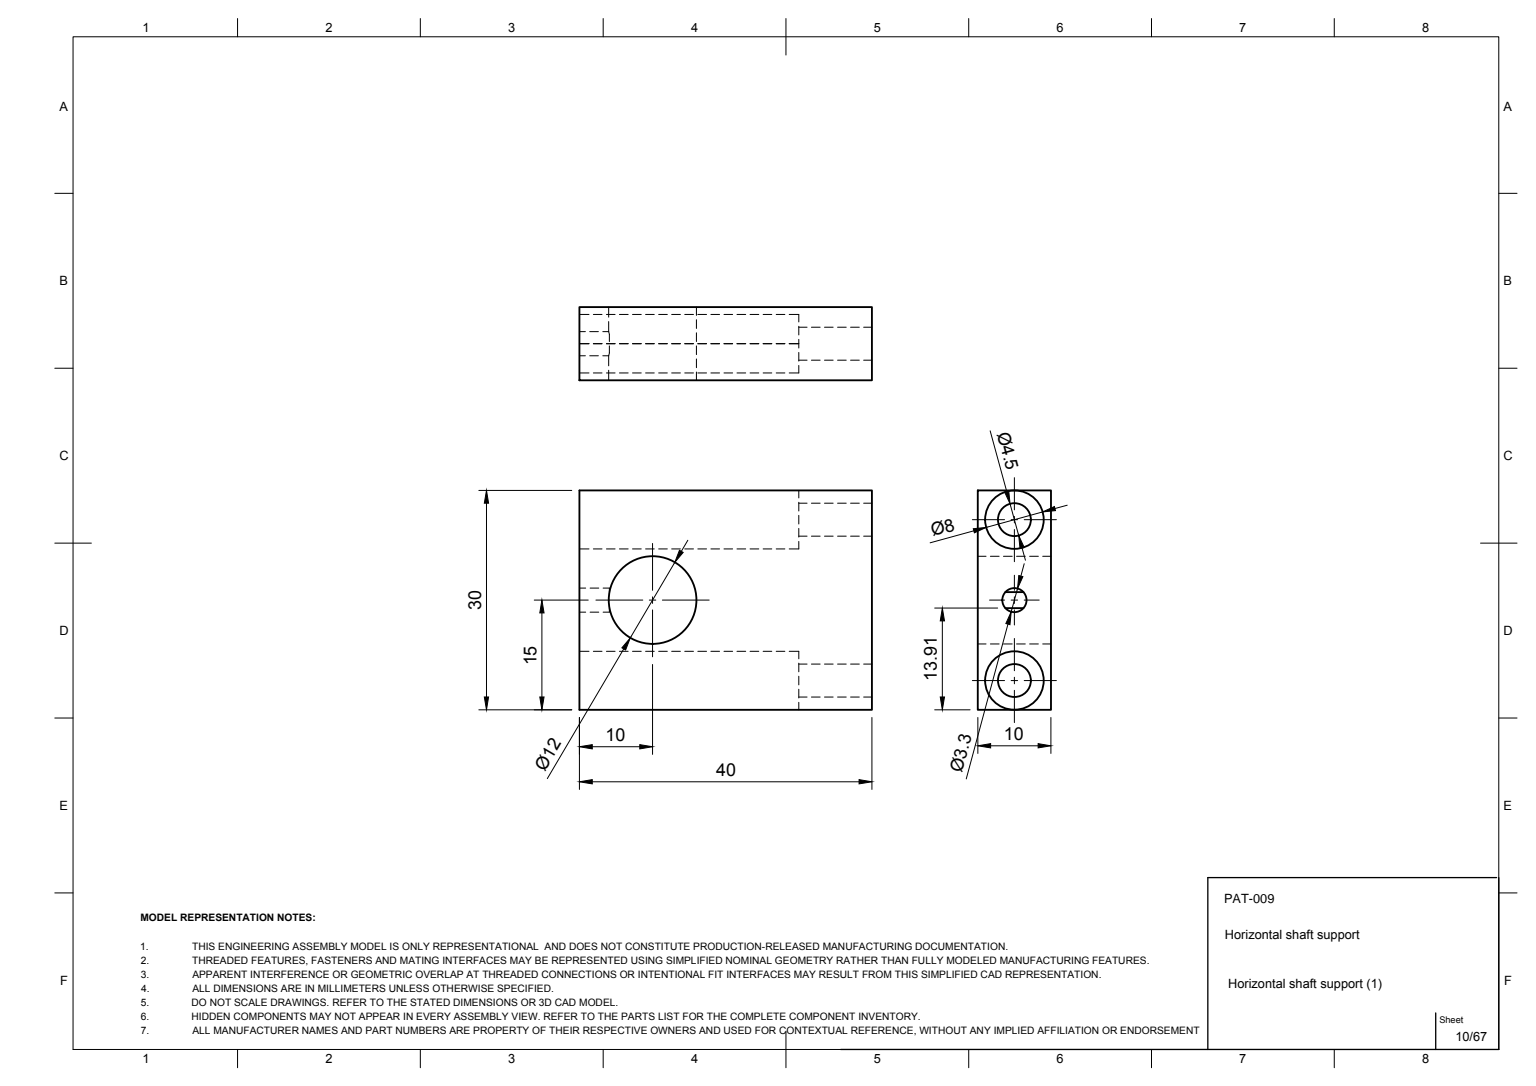
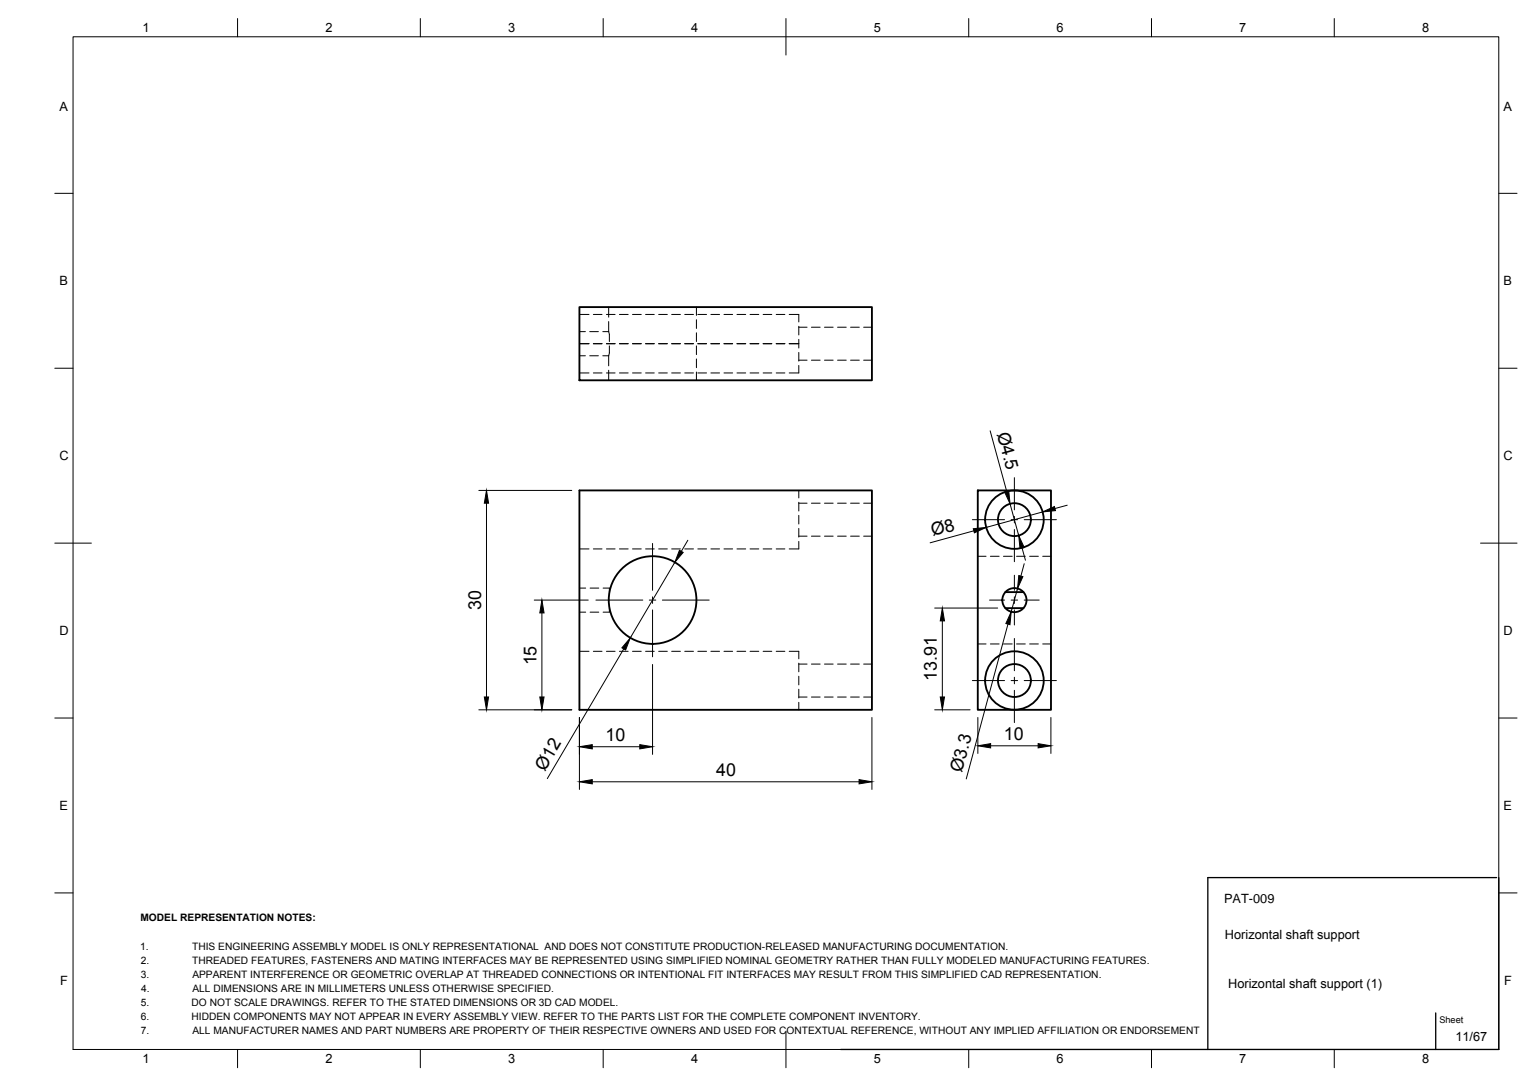
ISO-10303-21;
HEADER;
/* Generated by software containing ST-Developer
 * from STEP Tools, Inc. (www.steptools.com) 
 */

FILE_DESCRIPTION(
/* description */ ('Bell-crank linkage with push rods'),
/* implementation_level */ '2;1');

FILE_NAME(
/* name */ 'Horizontal shaft support.step',
/* time_stamp */ '2026-10-28T03:25:15-07:00',
/* author */ (''),
/* organization */ (''),
/* preprocessor_version */ 'ST-DEVELOPER v20.2',
/* originating_system */ 'Autodesk Translation Framework v15.17.0.0',
/* authorisation */ '');

FILE_SCHEMA (('AUTOMOTIVE_DESIGN { 1 0 10303 214 3 1 1 }'));
ENDSEC;

DATA;
#10=MECHANICAL_DESIGN_GEOMETRIC_PRESENTATION_REPRESENTATION('',(#609),#16678);
#461=B_SPLINE_CURVE_WITH_KNOTS('',3,(#13994,#13995,#13996,#13997,#13998,
#13999),.UNSPECIFIED.,.F.,.F.,(4,2,4),(0.635430324955934,0.687528937234029,
0.750024497760675),.UNSPECIFIED.);
#462=B_SPLINE_CURVE_WITH_KNOTS('',3,(#14003,#14004,#14005,#14006,#14007,
#14008),.UNSPECIFIED.,.F.,.F.,(4,2,4),(0.250008165920225,0.312503726446871,
0.364602338724967),.UNSPECIFIED.);
#463=B_SPLINE_CURVE_WITH_KNOTS('',3,(#14009,#14010,#14011,#14012,#14013,
#14014),.UNSPECIFIED.,.F.,.F.,(4,2,4),(0.135413993115484,0.187512605393579,
0.250008165920225),.UNSPECIFIED.);
#464=B_SPLINE_CURVE_WITH_KNOTS('',3,(#14015,#14016,#14017,#14018,#14019,
#14020),.UNSPECIFIED.,.F.,.F.,(4,2,4),(0.750024497760675,0.81252005828732,
0.864618670565416),.UNSPECIFIED.);
#501=SHAPE_REPRESENTATION_RELATIONSHIP('SRR','None',#16917,#555);
#555=ADVANCED_BREP_SHAPE_REPRESENTATION('',(#671),#16622);
#609=STYLED_ITEM('',(#17291),#671);
#671=MANIFOLD_SOLID_BREP('Body1',#8799);
#782=FACE_BOUND('',#1910,.T.);
#783=FACE_BOUND('',#1913,.T.);
#784=FACE_BOUND('',#1915,.T.);
#785=FACE_BOUND('',#1921,.T.);
#786=FACE_BOUND('',#1924,.T.);
#787=FACE_BOUND('',#1926,.T.);
#788=FACE_BOUND('',#1927,.T.);
#1003=PLANE('',#9631);
#1004=PLANE('',#9636);
#1005=PLANE('',#9640);
#1006=PLANE('',#9645);
#1007=PLANE('',#9647);
#1008=PLANE('',#9655);
#1009=PLANE('',#9656);
#1010=PLANE('',#9657);
#1011=PLANE('',#9658);
#1012=PLANE('',#9659);
#1324=FACE_OUTER_BOUND('',#1903,.T.);
#1325=FACE_OUTER_BOUND('',#1904,.T.);
#1326=FACE_OUTER_BOUND('',#1905,.T.);
#1327=FACE_OUTER_BOUND('',#1906,.T.);
#1328=FACE_OUTER_BOUND('',#1907,.T.);
#1329=FACE_OUTER_BOUND('',#1908,.T.);
#1330=FACE_OUTER_BOUND('',#1909,.T.);
#1331=FACE_OUTER_BOUND('',#1911,.T.);
#1332=FACE_OUTER_BOUND('',#1912,.T.);
#1333=FACE_OUTER_BOUND('',#1914,.T.);
#1334=FACE_OUTER_BOUND('',#1916,.T.);
#1335=FACE_OUTER_BOUND('',#1917,.T.);
#1336=FACE_OUTER_BOUND('',#1918,.T.);
#1337=FACE_OUTER_BOUND('',#1919,.T.);
#1338=FACE_OUTER_BOUND('',#1920,.T.);
#1339=FACE_OUTER_BOUND('',#1922,.T.);
#1340=FACE_OUTER_BOUND('',#1923,.T.);
#1341=FACE_OUTER_BOUND('',#1925,.T.);
#1903=EDGE_LOOP('',(#6251,#6252,#6253,#6254));
#1904=EDGE_LOOP('',(#6255,#6256,#6257,#6258));
#1905=EDGE_LOOP('',(#6259,#6260));
#1906=EDGE_LOOP('',(#6261,#6262,#6263,#6264,#6265,#6266,#6267,#6268,#6269));
#1907=EDGE_LOOP('',(#6270,#6271));
#1908=EDGE_LOOP('',(#6272,#6273,#6274,#6275));
#1909=EDGE_LOOP('',(#6276,#6277));
#1910=EDGE_LOOP('',(#6278));
#1911=EDGE_LOOP('',(#6279,#6280,#6281,#6282));
#1912=EDGE_LOOP('',(#6283,#6284));
#1913=EDGE_LOOP('',(#6285));
#1914=EDGE_LOOP('',(#6286,#6287,#6288,#6289,#6290,#6291,#6292,#6293,#6294,
#6295));
#1915=EDGE_LOOP('',(#6296));
#1916=EDGE_LOOP('',(#6297,#6298,#6299,#6300));
#1917=EDGE_LOOP('',(#6301,#6302,#6303,#6304));
#1918=EDGE_LOOP('',(#6305,#6306,#6307,#6308,#6309,#6310,#6311,#6312,#6313,
#6314,#6315,#6316));
#1919=EDGE_LOOP('',(#6317,#6318,#6319,#6320,#6321,#6322,#6323));
#1920=EDGE_LOOP('',(#6324,#6325,#6326,#6327));
#1921=EDGE_LOOP('',(#6328));
#1922=EDGE_LOOP('',(#6329,#6330,#6331,#6332,#6333,#6334,#6335));
#1923=EDGE_LOOP('',(#6336,#6337,#6338,#6339));
#1924=EDGE_LOOP('',(#6340));
#1925=EDGE_LOOP('',(#6341,#6342,#6343,#6344));
#1926=EDGE_LOOP('',(#6345));
#1927=EDGE_LOOP('',(#6346));
#2612=LINE('',#13971,#3161);
#2613=LINE('',#13975,#3162);
#2614=LINE('',#13980,#3163);
#2615=LINE('',#13984,#3164);
#2616=LINE('',#13989,#3165);
#2617=LINE('',#14022,#3166);
#2618=LINE('',#14025,#3167);
#2619=LINE('',#14028,#3168);
#2620=LINE('',#14035,#3169);
#2621=LINE('',#14043,#3170);
#2622=LINE('',#14044,#3171);
#2623=LINE('',#14046,#3172);
#2624=LINE('',#14048,#3173);
#2625=LINE('',#14049,#3174);
#2626=LINE('',#14050,#3175);
#2627=LINE('',#14054,#3176);
#2628=LINE('',#14058,#3177);
#2629=LINE('',#14062,#3178);
#2630=LINE('',#14064,#3179);
#2631=LINE('',#14069,#3180);
#2632=LINE('',#14070,#3181);
#2633=LINE('',#14071,#3182);
#2634=LINE('',#14074,#3183);
#2635=LINE('',#14075,#3184);
#2636=LINE('',#14078,#3185);
#2637=LINE('',#14079,#3186);
#2638=LINE('',#14081,#3187);
#3161=VECTOR('',#11054,0.4);
#3162=VECTOR('',#11057,1.);
#3163=VECTOR('',#11062,0.4);
#3164=VECTOR('',#11065,1.);
#3165=VECTOR('',#11070,1.);
#3166=VECTOR('',#11077,0.165);
#3167=VECTOR('',#11082,1.);
#3168=VECTOR('',#11087,1.);
#3169=VECTOR('',#11098,1.);
#3170=VECTOR('',#11107,1.);
#3171=VECTOR('',#11108,1.);
#3172=VECTOR('',#11109,1.);
#3173=VECTOR('',#11110,1.);
#3174=VECTOR('',#11111,1.);
#3175=VECTOR('',#11112,1.);
#3176=VECTOR('',#11117,0.225);
#3177=VECTOR('',#11122,0.225);
#3178=VECTOR('',#11127,0.6);
#3179=VECTOR('',#11128,0.6);
#3180=VECTOR('',#11133,1.);
#3181=VECTOR('',#11134,1.);
#3182=VECTOR('',#11135,1.);
#3183=VECTOR('',#11138,1.);
#3184=VECTOR('',#11139,1.);
#3185=VECTOR('',#11142,1.);
#3186=VECTOR('',#11143,1.);
#3187=VECTOR('',#11146,1.);
#3716=CIRCLE('',#9626,0.4);
#3717=CIRCLE('',#9627,0.4);
#3718=CIRCLE('',#9629,0.4);
#3719=CIRCLE('',#9630,0.4);
#3720=CIRCLE('',#9632,0.165);
#3721=CIRCLE('',#9634,0.165);
#3722=CIRCLE('',#9635,0.165);
#3723=CIRCLE('',#9638,0.4);
#3724=CIRCLE('',#9639,0.4);
#3725=CIRCLE('',#9641,0.225);
#3726=CIRCLE('',#9643,0.4);
#3727=CIRCLE('',#9644,0.4);
#3728=CIRCLE('',#9646,0.225);
#3729=CIRCLE('',#9649,0.225);
#3730=CIRCLE('',#9651,0.225);
#3731=CIRCLE('',#9653,0.6);
#3732=CIRCLE('',#9654,0.6);
#4234=VERTEX_POINT('',#13969);
#4235=VERTEX_POINT('',#13970);
#4236=VERTEX_POINT('',#13972);
#4237=VERTEX_POINT('',#13974);
#4238=VERTEX_POINT('',#13978);
#4239=VERTEX_POINT('',#13979);
#4240=VERTEX_POINT('',#13981);
#4241=VERTEX_POINT('',#13983);
#4242=VERTEX_POINT('',#13987);
#4243=VERTEX_POINT('',#13988);
#4244=VERTEX_POINT('',#13992);
#4245=VERTEX_POINT('',#13993);
#4246=VERTEX_POINT('',#14000);
#4247=VERTEX_POINT('',#14002);
#4248=VERTEX_POINT('',#14021);
#4249=VERTEX_POINT('',#14031);
#4250=VERTEX_POINT('',#14038);
#4251=VERTEX_POINT('',#14041);
#4252=VERTEX_POINT('',#14042);
#4253=VERTEX_POINT('',#14045);
#4254=VERTEX_POINT('',#14047);
#4255=VERTEX_POINT('',#14052);
#4256=VERTEX_POINT('',#14056);
#4257=VERTEX_POINT('',#14060);
#4258=VERTEX_POINT('',#14063);
#4259=VERTEX_POINT('',#14067);
#4260=VERTEX_POINT('',#14068);
#4261=VERTEX_POINT('',#14073);
#4262=VERTEX_POINT('',#14077);
#5003=EDGE_CURVE('',#4234,#4235,#2612,.T.);
#5004=EDGE_CURVE('',#4236,#4234,#3716,.T.);
#5005=EDGE_CURVE('',#4236,#4237,#2613,.T.);
#5006=EDGE_CURVE('',#4235,#4237,#3717,.T.);
#5007=EDGE_CURVE('',#4238,#4239,#2614,.T.);
#5008=EDGE_CURVE('',#4240,#4238,#3718,.T.);
#5009=EDGE_CURVE('',#4240,#4241,#2615,.T.);
#5010=EDGE_CURVE('',#4239,#4241,#3719,.T.);
#5011=EDGE_CURVE('',#4242,#4243,#2616,.T.);
#5012=EDGE_CURVE('',#4242,#4243,#3720,.T.);
#5013=EDGE_CURVE('',#4244,#4245,#461,.T.);
#5014=EDGE_CURVE('',#4246,#4244,#3721,.T.);
#5015=EDGE_CURVE('',#4247,#4246,#462,.T.);
#5016=EDGE_CURVE('',#4243,#4247,#463,.T.);
#5017=EDGE_CURVE('',#4245,#4242,#464,.T.);
#5018=EDGE_CURVE('',#4245,#4248,#2617,.T.);
#5019=EDGE_CURVE('',#4248,#4248,#3722,.T.);
#5020=EDGE_CURVE('',#4246,#4244,#2618,.T.);
#5021=EDGE_CURVE('',#4241,#4239,#3723,.T.);
#5022=EDGE_CURVE('',#4240,#4241,#2619,.T.);
#5023=EDGE_CURVE('',#4238,#4240,#3724,.T.);
#5024=EDGE_CURVE('',#4249,#4249,#3725,.T.);
#5025=EDGE_CURVE('',#4237,#4235,#3726,.T.);
#5026=EDGE_CURVE('',#4236,#4237,#2620,.T.);
#5027=EDGE_CURVE('',#4234,#4236,#3727,.T.);
#5028=EDGE_CURVE('',#4250,#4250,#3728,.T.);
#5029=EDGE_CURVE('',#4251,#4252,#2621,.T.);
#5030=EDGE_CURVE('',#4252,#4241,#2622,.T.);
#5031=EDGE_CURVE('',#4241,#4253,#2623,.T.);
#5032=EDGE_CURVE('',#4253,#4254,#2624,.T.);
#5033=EDGE_CURVE('',#4254,#4237,#2625,.T.);
#5034=EDGE_CURVE('',#4237,#4251,#2626,.T.);
#5035=EDGE_CURVE('',#4255,#4255,#3729,.T.);
#5036=EDGE_CURVE('',#4255,#4249,#2627,.T.);
#5037=EDGE_CURVE('',#4256,#4256,#3730,.T.);
#5038=EDGE_CURVE('',#4256,#4250,#2628,.T.);
#5039=EDGE_CURVE('',#4257,#4257,#3731,.T.);
#5040=EDGE_CURVE('',#4257,#4245,#2629,.T.);
#5041=EDGE_CURVE('',#4247,#4258,#2630,.T.);
#5042=EDGE_CURVE('',#4258,#4258,#3732,.T.);
#5043=EDGE_CURVE('',#4259,#4260,#2631,.T.);
#5044=EDGE_CURVE('',#4260,#4251,#2632,.T.);
#5045=EDGE_CURVE('',#4259,#4254,#2633,.T.);
#5046=EDGE_CURVE('',#4261,#4259,#2634,.T.);
#5047=EDGE_CURVE('',#4261,#4253,#2635,.T.);
#5048=EDGE_CURVE('',#4262,#4261,#2636,.T.);
#5049=EDGE_CURVE('',#4262,#4252,#2637,.T.);
#5050=EDGE_CURVE('',#4260,#4262,#2638,.T.);
#6251=ORIENTED_EDGE('',*,*,#5003,.F.);
#6252=ORIENTED_EDGE('',*,*,#5004,.F.);
#6253=ORIENTED_EDGE('',*,*,#5005,.T.);
#6254=ORIENTED_EDGE('',*,*,#5006,.F.);
#6255=ORIENTED_EDGE('',*,*,#5007,.F.);
#6256=ORIENTED_EDGE('',*,*,#5008,.F.);
#6257=ORIENTED_EDGE('',*,*,#5009,.T.);
#6258=ORIENTED_EDGE('',*,*,#5010,.F.);
#6259=ORIENTED_EDGE('',*,*,#5011,.F.);
#6260=ORIENTED_EDGE('',*,*,#5012,.T.);
#6261=ORIENTED_EDGE('',*,*,#5013,.F.);
#6262=ORIENTED_EDGE('',*,*,#5014,.F.);
#6263=ORIENTED_EDGE('',*,*,#5015,.F.);
#6264=ORIENTED_EDGE('',*,*,#5016,.F.);
#6265=ORIENTED_EDGE('',*,*,#5012,.F.);
#6266=ORIENTED_EDGE('',*,*,#5017,.F.);
#6267=ORIENTED_EDGE('',*,*,#5018,.T.);
#6268=ORIENTED_EDGE('',*,*,#5019,.F.);
#6269=ORIENTED_EDGE('',*,*,#5018,.F.);
#6270=ORIENTED_EDGE('',*,*,#5020,.F.);
#6271=ORIENTED_EDGE('',*,*,#5014,.T.);
#6272=ORIENTED_EDGE('',*,*,#5007,.T.);
#6273=ORIENTED_EDGE('',*,*,#5021,.F.);
#6274=ORIENTED_EDGE('',*,*,#5022,.F.);
#6275=ORIENTED_EDGE('',*,*,#5023,.F.);
#6276=ORIENTED_EDGE('',*,*,#5008,.T.);
#6277=ORIENTED_EDGE('',*,*,#5023,.T.);
#6278=ORIENTED_EDGE('',*,*,#5024,.F.);
#6279=ORIENTED_EDGE('',*,*,#5003,.T.);
#6280=ORIENTED_EDGE('',*,*,#5025,.F.);
#6281=ORIENTED_EDGE('',*,*,#5026,.F.);
#6282=ORIENTED_EDGE('',*,*,#5027,.F.);
#6283=ORIENTED_EDGE('',*,*,#5004,.T.);
#6284=ORIENTED_EDGE('',*,*,#5027,.T.);
#6285=ORIENTED_EDGE('',*,*,#5028,.F.);
#6286=ORIENTED_EDGE('',*,*,#5029,.T.);
#6287=ORIENTED_EDGE('',*,*,#5030,.T.);
#6288=ORIENTED_EDGE('',*,*,#5021,.T.);
#6289=ORIENTED_EDGE('',*,*,#5010,.T.);
#6290=ORIENTED_EDGE('',*,*,#5031,.T.);
#6291=ORIENTED_EDGE('',*,*,#5032,.T.);
#6292=ORIENTED_EDGE('',*,*,#5033,.T.);
#6293=ORIENTED_EDGE('',*,*,#5025,.T.);
#6294=ORIENTED_EDGE('',*,*,#5006,.T.);
#6295=ORIENTED_EDGE('',*,*,#5034,.T.);
#6296=ORIENTED_EDGE('',*,*,#5019,.T.);
#6297=ORIENTED_EDGE('',*,*,#5035,.F.);
#6298=ORIENTED_EDGE('',*,*,#5036,.T.);
#6299=ORIENTED_EDGE('',*,*,#5024,.T.);
#6300=ORIENTED_EDGE('',*,*,#5036,.F.);
#6301=ORIENTED_EDGE('',*,*,#5037,.F.);
#6302=ORIENTED_EDGE('',*,*,#5038,.T.);
#6303=ORIENTED_EDGE('',*,*,#5028,.T.);
#6304=ORIENTED_EDGE('',*,*,#5038,.F.);
#6305=ORIENTED_EDGE('',*,*,#5039,.F.);
#6306=ORIENTED_EDGE('',*,*,#5040,.T.);
#6307=ORIENTED_EDGE('',*,*,#5017,.T.);
#6308=ORIENTED_EDGE('',*,*,#5011,.T.);
#6309=ORIENTED_EDGE('',*,*,#5016,.T.);
#6310=ORIENTED_EDGE('',*,*,#5041,.T.);
#6311=ORIENTED_EDGE('',*,*,#5042,.F.);
#6312=ORIENTED_EDGE('',*,*,#5041,.F.);
#6313=ORIENTED_EDGE('',*,*,#5015,.T.);
#6314=ORIENTED_EDGE('',*,*,#5020,.T.);
#6315=ORIENTED_EDGE('',*,*,#5013,.T.);
#6316=ORIENTED_EDGE('',*,*,#5040,.F.);
#6317=ORIENTED_EDGE('',*,*,#5043,.T.);
#6318=ORIENTED_EDGE('',*,*,#5044,.T.);
#6319=ORIENTED_EDGE('',*,*,#5034,.F.);
#6320=ORIENTED_EDGE('',*,*,#5005,.F.);
#6321=ORIENTED_EDGE('',*,*,#5026,.T.);
#6322=ORIENTED_EDGE('',*,*,#5033,.F.);
#6323=ORIENTED_EDGE('',*,*,#5045,.F.);
#6324=ORIENTED_EDGE('',*,*,#5046,.T.);
#6325=ORIENTED_EDGE('',*,*,#5045,.T.);
#6326=ORIENTED_EDGE('',*,*,#5032,.F.);
#6327=ORIENTED_EDGE('',*,*,#5047,.F.);
#6328=ORIENTED_EDGE('',*,*,#5042,.T.);
#6329=ORIENTED_EDGE('',*,*,#5048,.T.);
#6330=ORIENTED_EDGE('',*,*,#5047,.T.);
#6331=ORIENTED_EDGE('',*,*,#5031,.F.);
#6332=ORIENTED_EDGE('',*,*,#5009,.F.);
#6333=ORIENTED_EDGE('',*,*,#5022,.T.);
#6334=ORIENTED_EDGE('',*,*,#5030,.F.);
#6335=ORIENTED_EDGE('',*,*,#5049,.F.);
#6336=ORIENTED_EDGE('',*,*,#5050,.T.);
#6337=ORIENTED_EDGE('',*,*,#5049,.T.);
#6338=ORIENTED_EDGE('',*,*,#5029,.F.);
#6339=ORIENTED_EDGE('',*,*,#5044,.F.);
#6340=ORIENTED_EDGE('',*,*,#5039,.T.);
#6341=ORIENTED_EDGE('',*,*,#5050,.F.);
#6342=ORIENTED_EDGE('',*,*,#5043,.F.);
#6343=ORIENTED_EDGE('',*,*,#5046,.F.);
#6344=ORIENTED_EDGE('',*,*,#5048,.F.);
#6345=ORIENTED_EDGE('',*,*,#5035,.T.);
#6346=ORIENTED_EDGE('',*,*,#5037,.T.);
#8107=CYLINDRICAL_SURFACE('',#9625,0.4);
#8108=CYLINDRICAL_SURFACE('',#9628,0.4);
#8109=CYLINDRICAL_SURFACE('',#9633,0.165);
#8110=CYLINDRICAL_SURFACE('',#9637,0.4);
#8111=CYLINDRICAL_SURFACE('',#9642,0.4);
#8112=CYLINDRICAL_SURFACE('',#9648,0.225);
#8113=CYLINDRICAL_SURFACE('',#9650,0.225);
#8114=CYLINDRICAL_SURFACE('',#9652,0.6);
#8349=ADVANCED_FACE('',(#1324),#8107,.F.);
#8350=ADVANCED_FACE('',(#1325),#8108,.F.);
#8351=ADVANCED_FACE('',(#1326),#1003,.T.);
#8352=ADVANCED_FACE('',(#1327),#8109,.F.);
#8353=ADVANCED_FACE('',(#1328),#1004,.T.);
#8354=ADVANCED_FACE('',(#1329),#8110,.F.);
#8355=ADVANCED_FACE('',(#1330,#782),#1005,.T.);
#8356=ADVANCED_FACE('',(#1331),#8111,.F.);
#8357=ADVANCED_FACE('',(#1332,#783),#1006,.T.);
#8358=ADVANCED_FACE('',(#1333,#784),#1007,.T.);
#8359=ADVANCED_FACE('',(#1334),#8112,.F.);
#8360=ADVANCED_FACE('',(#1335),#8113,.F.);
#8361=ADVANCED_FACE('',(#1336),#8114,.F.);
#8362=ADVANCED_FACE('',(#1337),#1008,.T.);
#8363=ADVANCED_FACE('',(#1338,#785),#1009,.T.);
#8364=ADVANCED_FACE('',(#1339),#1010,.T.);
#8365=ADVANCED_FACE('',(#1340,#786),#1011,.T.);
#8366=ADVANCED_FACE('',(#1341,#787,#788),#1012,.F.);
#8799=CLOSED_SHELL('',(#8349,#8350,#8351,#8352,#8353,#8354,#8355,#8356,
#8357,#8358,#8359,#8360,#8361,#8362,#8363,#8364,#8365,#8366));
#9624=AXIS2_PLACEMENT_3D('',#13967,#11050,#11051);
#9625=AXIS2_PLACEMENT_3D('',#13968,#11052,#11053);
#9626=AXIS2_PLACEMENT_3D('',#13973,#11055,#11056);
#9627=AXIS2_PLACEMENT_3D('',#13976,#11058,#11059);
#9628=AXIS2_PLACEMENT_3D('',#13977,#11060,#11061);
#9629=AXIS2_PLACEMENT_3D('',#13982,#11063,#11064);
#9630=AXIS2_PLACEMENT_3D('',#13985,#11066,#11067);
#9631=AXIS2_PLACEMENT_3D('',#13986,#11068,#11069);
#9632=AXIS2_PLACEMENT_3D('',#13990,#11071,#11072);
#9633=AXIS2_PLACEMENT_3D('',#13991,#11073,#11074);
#9634=AXIS2_PLACEMENT_3D('',#14001,#11075,#11076);
#9635=AXIS2_PLACEMENT_3D('',#14023,#11078,#11079);
#9636=AXIS2_PLACEMENT_3D('',#14024,#11080,#11081);
#9637=AXIS2_PLACEMENT_3D('',#14026,#11083,#11084);
#9638=AXIS2_PLACEMENT_3D('',#14027,#11085,#11086);
#9639=AXIS2_PLACEMENT_3D('',#14029,#11088,#11089);
#9640=AXIS2_PLACEMENT_3D('',#14030,#11090,#11091);
#9641=AXIS2_PLACEMENT_3D('',#14032,#11092,#11093);
#9642=AXIS2_PLACEMENT_3D('',#14033,#11094,#11095);
#9643=AXIS2_PLACEMENT_3D('',#14034,#11096,#11097);
#9644=AXIS2_PLACEMENT_3D('',#14036,#11099,#11100);
#9645=AXIS2_PLACEMENT_3D('',#14037,#11101,#11102);
#9646=AXIS2_PLACEMENT_3D('',#14039,#11103,#11104);
#9647=AXIS2_PLACEMENT_3D('',#14040,#11105,#11106);
#9648=AXIS2_PLACEMENT_3D('',#14051,#11113,#11114);
#9649=AXIS2_PLACEMENT_3D('',#14053,#11115,#11116);
#9650=AXIS2_PLACEMENT_3D('',#14055,#11118,#11119);
#9651=AXIS2_PLACEMENT_3D('',#14057,#11120,#11121);
#9652=AXIS2_PLACEMENT_3D('',#14059,#11123,#11124);
#9653=AXIS2_PLACEMENT_3D('',#14061,#11125,#11126);
#9654=AXIS2_PLACEMENT_3D('',#14065,#11129,#11130);
#9655=AXIS2_PLACEMENT_3D('',#14066,#11131,#11132);
#9656=AXIS2_PLACEMENT_3D('',#14072,#11136,#11137);
#9657=AXIS2_PLACEMENT_3D('',#14076,#11140,#11141);
#9658=AXIS2_PLACEMENT_3D('',#14080,#11144,#11145);
#9659=AXIS2_PLACEMENT_3D('',#14082,#11147,#11148);
#11050=DIRECTION('axis',(0.,0.,1.));
#11051=DIRECTION('refdir',(1.,0.,0.));
#11052=DIRECTION('center_axis',(0.,0.,1.));
#11053=DIRECTION('ref_axis',(1.,0.,0.));
#11054=DIRECTION('',(0.,0.,1.));
#11055=DIRECTION('center_axis',(0.,0.,1.));
#11056=DIRECTION('ref_axis',(1.,0.,0.));
#11057=DIRECTION('',(0.,0.,1.));
#11058=DIRECTION('center_axis',(0.,0.,-1.));
#11059=DIRECTION('ref_axis',(1.,0.,0.));
#11060=DIRECTION('center_axis',(0.,0.,1.));
#11061=DIRECTION('ref_axis',(1.,0.,0.));
#11062=DIRECTION('',(0.,0.,1.));
#11063=DIRECTION('center_axis',(0.,0.,1.));
#11064=DIRECTION('ref_axis',(1.,0.,0.));
#11065=DIRECTION('',(0.,0.,1.));
#11066=DIRECTION('center_axis',(0.,0.,-1.));
#11067=DIRECTION('ref_axis',(1.,0.,0.));
#11068=DIRECTION('center_axis',(0.,0.,1.));
#11069=DIRECTION('ref_axis',(1.,0.,0.));
#11070=DIRECTION('',(1.,0.,0.));
#11071=DIRECTION('center_axis',(0.,0.,1.));
#11072=DIRECTION('ref_axis',(1.,0.,0.));
#11073=DIRECTION('center_axis',(0.,0.,1.));
#11074=DIRECTION('ref_axis',(1.,0.,0.));
#11075=DIRECTION('center_axis',(0.,0.,1.));
#11076=DIRECTION('ref_axis',(1.,0.,0.));
#11077=DIRECTION('',(0.,0.,1.));
#11078=DIRECTION('center_axis',(0.,0.,-1.));
#11079=DIRECTION('ref_axis',(1.,0.,0.));
#11080=DIRECTION('center_axis',(0.,0.,1.));
#11081=DIRECTION('ref_axis',(1.,0.,0.));
#11082=DIRECTION('',(-1.,0.,0.));
#11083=DIRECTION('center_axis',(0.,0.,1.));
#11084=DIRECTION('ref_axis',(1.,0.,0.));
#11085=DIRECTION('center_axis',(0.,0.,-1.));
#11086=DIRECTION('ref_axis',(1.,0.,0.));
#11087=DIRECTION('',(0.,0.,1.));
#11088=DIRECTION('center_axis',(0.,0.,1.));
#11089=DIRECTION('ref_axis',(1.,0.,0.));
#11090=DIRECTION('center_axis',(0.,0.,1.));
#11091=DIRECTION('ref_axis',(1.,0.,0.));
#11092=DIRECTION('center_axis',(0.,0.,1.));
#11093=DIRECTION('ref_axis',(1.,0.,0.));
#11094=DIRECTION('center_axis',(0.,0.,1.));
#11095=DIRECTION('ref_axis',(1.,0.,0.));
#11096=DIRECTION('center_axis',(0.,0.,-1.));
#11097=DIRECTION('ref_axis',(1.,0.,0.));
#11098=DIRECTION('',(0.,0.,1.));
#11099=DIRECTION('center_axis',(0.,0.,1.));
#11100=DIRECTION('ref_axis',(1.,0.,0.));
#11101=DIRECTION('center_axis',(0.,0.,1.));
#11102=DIRECTION('ref_axis',(1.,0.,0.));
#11103=DIRECTION('center_axis',(0.,0.,1.));
#11104=DIRECTION('ref_axis',(1.,0.,0.));
#11105=DIRECTION('center_axis',(0.,0.,1.));
#11106=DIRECTION('ref_axis',(1.,0.,0.));
#11107=DIRECTION('',(0.,-1.,0.));
#11108=DIRECTION('',(1.,0.,0.));
#11109=DIRECTION('',(1.,0.,0.));
#11110=DIRECTION('',(0.,1.,0.));
#11111=DIRECTION('',(-1.,0.,0.));
#11112=DIRECTION('',(-1.,0.,0.));
#11113=DIRECTION('center_axis',(0.,0.,1.));
#11114=DIRECTION('ref_axis',(1.,0.,0.));
#11115=DIRECTION('center_axis',(0.,0.,1.));
#11116=DIRECTION('ref_axis',(1.,0.,0.));
#11117=DIRECTION('',(0.,0.,1.));
#11118=DIRECTION('center_axis',(0.,0.,1.));
#11119=DIRECTION('ref_axis',(1.,0.,0.));
#11120=DIRECTION('center_axis',(0.,0.,1.));
#11121=DIRECTION('ref_axis',(1.,0.,0.));
#11122=DIRECTION('',(0.,0.,1.));
#11123=DIRECTION('center_axis',(1.,0.,0.));
#11124=DIRECTION('ref_axis',(0.,0.,-1.));
#11125=DIRECTION('center_axis',(1.,0.,0.));
#11126=DIRECTION('ref_axis',(0.,0.,-1.));
#11127=DIRECTION('',(1.,0.,0.));
#11128=DIRECTION('',(1.,0.,0.));
#11129=DIRECTION('center_axis',(-1.,0.,0.));
#11130=DIRECTION('ref_axis',(0.,0.,-1.));
#11131=DIRECTION('center_axis',(0.,1.,0.));
#11132=DIRECTION('ref_axis',(-1.,0.,0.));
#11133=DIRECTION('',(-1.,0.,0.));
#11134=DIRECTION('',(0.,0.,1.));
#11135=DIRECTION('',(0.,0.,1.));
#11136=DIRECTION('center_axis',(1.,0.,0.));
#11137=DIRECTION('ref_axis',(0.,1.,0.));
#11138=DIRECTION('',(0.,1.,0.));
#11139=DIRECTION('',(0.,0.,1.));
#11140=DIRECTION('center_axis',(0.,-1.,0.));
#11141=DIRECTION('ref_axis',(1.,0.,0.));
#11142=DIRECTION('',(1.,0.,0.));
#11143=DIRECTION('',(0.,0.,1.));
#11144=DIRECTION('center_axis',(-1.,0.,0.));
#11145=DIRECTION('ref_axis',(0.,-1.,0.));
#11146=DIRECTION('',(0.,-1.,0.));
#11147=DIRECTION('center_axis',(0.,0.,1.));
#11148=DIRECTION('ref_axis',(1.,0.,0.));
#13967=CARTESIAN_POINT('',(0.,0.,0.));
#13968=CARTESIAN_POINT('Origin',(5.5,3.1,2.));
#13969=CARTESIAN_POINT('',(5.1,3.1,2.));
#13970=CARTESIAN_POINT('',(5.1,3.1,5.));
#13971=CARTESIAN_POINT('',(5.1,3.1,2.));
#13972=CARTESIAN_POINT('',(5.5,3.5,2.));
#13973=CARTESIAN_POINT('Origin',(5.5,3.1,2.));
#13974=CARTESIAN_POINT('',(5.5,3.5,5.));
#13975=CARTESIAN_POINT('',(5.5,3.5,2.));
#13976=CARTESIAN_POINT('Origin',(5.5,3.1,5.));
#13977=CARTESIAN_POINT('Origin',(5.5,0.9,2.));
#13978=CARTESIAN_POINT('',(5.1,0.9,2.));
#13979=CARTESIAN_POINT('',(5.1,0.9,5.));
#13980=CARTESIAN_POINT('',(5.1,0.9,2.));
#13981=CARTESIAN_POINT('',(5.5,0.5,2.));
#13982=CARTESIAN_POINT('Origin',(5.5,0.9,2.));
#13983=CARTESIAN_POINT('',(5.5,0.5,5.));
#13984=CARTESIAN_POINT('',(5.5,0.5,2.));
#13985=CARTESIAN_POINT('Origin',(5.5,0.9,5.));
#13986=CARTESIAN_POINT('Origin',(5.5,2.,4.59));
#13987=CARTESIAN_POINT('',(5.3762058159686,1.89091287885364,4.59));
#13988=CARTESIAN_POINT('',(5.6237941840314,1.89091287885364,4.59));
#13989=CARTESIAN_POINT('',(4.9,1.89091287885364,4.59));
#13990=CARTESIAN_POINT('Origin',(5.5,2.,4.59));
#13991=CARTESIAN_POINT('Origin',(5.5,2.,4.59));
#13992=CARTESIAN_POINT('',(5.3762058159686,2.10908712114636,4.59));
#13993=CARTESIAN_POINT('',(5.335,2.,4.6));
#13994=CARTESIAN_POINT('Ctrl Pts',(5.3762058159686,2.10908712114636,4.59));
#13995=CARTESIAN_POINT('Ctrl Pts',(5.36460086481047,2.09591759715261,4.59243495840567));
#13996=CARTESIAN_POINT('Ctrl Pts',(5.35465435634175,2.08022344943772,4.59485638705045));
#13997=CARTESIAN_POINT('Ctrl Pts',(5.33918513536598,2.04298016596019,4.59880705606552));
#13998=CARTESIAN_POINT('Ctrl Pts',(5.335,2.02083185350888,4.6));
#13999=CARTESIAN_POINT('Ctrl Pts',(5.335,2.,4.6));
#14000=CARTESIAN_POINT('',(5.6237941840314,2.10908712114636,4.59));
#14001=CARTESIAN_POINT('Origin',(5.5,2.,4.59));
#14002=CARTESIAN_POINT('',(5.665,2.,4.6));
#14003=CARTESIAN_POINT('Ctrl Pts',(5.665,2.,4.6));
#14004=CARTESIAN_POINT('Ctrl Pts',(5.665,2.02083185350888,4.6));
#14005=CARTESIAN_POINT('Ctrl Pts',(5.66081486463402,2.04298016596019,4.59880705606552));
#14006=CARTESIAN_POINT('Ctrl Pts',(5.64534564365825,2.08022344943772,4.59485638705045));
#14007=CARTESIAN_POINT('Ctrl Pts',(5.63539913518953,2.09591759715261,4.59243495840567));
#14008=CARTESIAN_POINT('Ctrl Pts',(5.6237941840314,2.10908712114636,4.59));
#14009=CARTESIAN_POINT('Ctrl Pts',(5.6237941840314,1.89091287885364,4.59));
#14010=CARTESIAN_POINT('Ctrl Pts',(5.63539913518953,1.90408240284739,4.59243495840567));
#14011=CARTESIAN_POINT('Ctrl Pts',(5.64534564365825,1.91977655056228,4.59485638705045));
#14012=CARTESIAN_POINT('Ctrl Pts',(5.66081486463402,1.95701983403981,4.59880705606552));
#14013=CARTESIAN_POINT('Ctrl Pts',(5.665,1.97916814649112,4.6));
#14014=CARTESIAN_POINT('Ctrl Pts',(5.665,2.,4.6));
#14015=CARTESIAN_POINT('Ctrl Pts',(5.335,2.,4.6));
#14016=CARTESIAN_POINT('Ctrl Pts',(5.335,1.97916814649112,4.6));
#14017=CARTESIAN_POINT('Ctrl Pts',(5.33918513536598,1.95701983403981,4.59880705606552));
#14018=CARTESIAN_POINT('Ctrl Pts',(5.35465435634175,1.91977655056228,4.59485638705045));
#14019=CARTESIAN_POINT('Ctrl Pts',(5.36460086481047,1.90408240284739,4.59243495840567));
#14020=CARTESIAN_POINT('Ctrl Pts',(5.3762058159686,1.89091287885364,4.59));
#14021=CARTESIAN_POINT('',(5.335,2.,5.));
#14022=CARTESIAN_POINT('',(5.335,2.,4.59));
#14023=CARTESIAN_POINT('Origin',(5.5,2.,5.));
#14024=CARTESIAN_POINT('Origin',(5.5,2.,4.59));
#14025=CARTESIAN_POINT('',(4.9,2.10908712114636,4.59));
#14026=CARTESIAN_POINT('Origin',(5.5,0.9,2.));
#14027=CARTESIAN_POINT('Origin',(5.5,0.9,5.));
#14028=CARTESIAN_POINT('',(5.5,0.5,2.));
#14029=CARTESIAN_POINT('Origin',(5.5,0.9,2.));
#14030=CARTESIAN_POINT('Origin',(5.5,0.9,2.));
#14031=CARTESIAN_POINT('',(5.275,0.9,2.));
#14032=CARTESIAN_POINT('Origin',(5.5,0.9,2.));
#14033=CARTESIAN_POINT('Origin',(5.5,3.1,2.));
#14034=CARTESIAN_POINT('Origin',(5.5,3.1,5.));
#14035=CARTESIAN_POINT('',(5.5,3.5,2.));
#14036=CARTESIAN_POINT('Origin',(5.5,3.1,2.));
#14037=CARTESIAN_POINT('Origin',(5.5,3.1,2.));
#14038=CARTESIAN_POINT('',(5.275,3.1,2.));
#14039=CARTESIAN_POINT('Origin',(5.5,3.1,2.));
#14040=CARTESIAN_POINT('Origin',(5.5,2.,5.));
#14041=CARTESIAN_POINT('',(5.,3.5,5.));
#14042=CARTESIAN_POINT('',(5.,0.5,5.));
#14043=CARTESIAN_POINT('',(5.,3.5,5.));
#14044=CARTESIAN_POINT('',(5.,0.5,5.));
#14045=CARTESIAN_POINT('',(6.,0.5,5.));
#14046=CARTESIAN_POINT('',(5.,0.5,5.));
#14047=CARTESIAN_POINT('',(6.,3.5,5.));
#14048=CARTESIAN_POINT('',(6.,0.5,5.));
#14049=CARTESIAN_POINT('',(6.,3.5,5.));
#14050=CARTESIAN_POINT('',(6.,3.5,5.));
#14051=CARTESIAN_POINT('Origin',(5.5,0.9,0.9));
#14052=CARTESIAN_POINT('',(5.275,0.9,1.));
#14053=CARTESIAN_POINT('Origin',(5.5,0.9,1.));
#14054=CARTESIAN_POINT('',(5.275,0.9,0.9));
#14055=CARTESIAN_POINT('Origin',(5.5,3.1,0.9));
#14056=CARTESIAN_POINT('',(5.275,3.1,1.));
#14057=CARTESIAN_POINT('Origin',(5.5,3.1,1.));
#14058=CARTESIAN_POINT('',(5.275,3.1,0.9));
#14059=CARTESIAN_POINT('Origin',(4.9,2.,4.));
#14060=CARTESIAN_POINT('',(5.,2.,4.6));
#14061=CARTESIAN_POINT('Origin',(5.,2.,4.));
#14062=CARTESIAN_POINT('',(4.9,2.,4.6));
#14063=CARTESIAN_POINT('',(6.,2.,4.6));
#14064=CARTESIAN_POINT('',(4.9,2.,4.6));
#14065=CARTESIAN_POINT('Origin',(6.,2.,4.));
#14066=CARTESIAN_POINT('Origin',(6.,3.5,1.));
#14067=CARTESIAN_POINT('',(6.,3.5,1.));
#14068=CARTESIAN_POINT('',(5.,3.5,1.));
#14069=CARTESIAN_POINT('',(6.,3.5,1.));
#14070=CARTESIAN_POINT('',(5.,3.5,1.));
#14071=CARTESIAN_POINT('',(6.,3.5,1.));
#14072=CARTESIAN_POINT('Origin',(6.,0.5,1.));
#14073=CARTESIAN_POINT('',(6.,0.5,1.));
#14074=CARTESIAN_POINT('',(6.,0.5,1.));
#14075=CARTESIAN_POINT('',(6.,0.5,1.));
#14076=CARTESIAN_POINT('Origin',(5.,0.5,1.));
#14077=CARTESIAN_POINT('',(5.,0.5,1.));
#14078=CARTESIAN_POINT('',(5.,0.5,1.));
#14079=CARTESIAN_POINT('',(5.,0.5,1.));
#14080=CARTESIAN_POINT('Origin',(5.,3.5,1.));
#14081=CARTESIAN_POINT('',(5.,3.5,1.));
#14082=CARTESIAN_POINT('Origin',(5.5,2.,1.));
#16558=UNCERTAINTY_MEASURE_WITH_UNIT(LENGTH_MEASURE(0.001),#16679,
'DISTANCE_ACCURACY_VALUE',
'Maximum model space distance between geometric entities at asserted c
onnectivities');
#16614=UNCERTAINTY_MEASURE_WITH_UNIT(LENGTH_MEASURE(0.001),#16679,
'DISTANCE_ACCURACY_VALUE',
'Maximum model space distance between geometric entities at asserted c
onnectivities');
#16622=(
GEOMETRIC_REPRESENTATION_CONTEXT(3)
GLOBAL_UNCERTAINTY_ASSIGNED_CONTEXT((#16558))
GLOBAL_UNIT_ASSIGNED_CONTEXT((#16679,#16681,#16682))
REPRESENTATION_CONTEXT('','3D')
);
#16678=(
GEOMETRIC_REPRESENTATION_CONTEXT(3)
GLOBAL_UNCERTAINTY_ASSIGNED_CONTEXT((#16614))
GLOBAL_UNIT_ASSIGNED_CONTEXT((#16679,#16681,#16682))
REPRESENTATION_CONTEXT('','3D')
);
#16679=(
LENGTH_UNIT()
NAMED_UNIT(*)
SI_UNIT(.CENTI.,.METRE.)
);
#16681=(
NAMED_UNIT(*)
PLANE_ANGLE_UNIT()
SI_UNIT($,.RADIAN.)
);
#16682=(
NAMED_UNIT(*)
SI_UNIT($,.STERADIAN.)
SOLID_ANGLE_UNIT()
);
#16690=SHAPE_DEFINITION_REPRESENTATION(#16753,#16917);
#16753=PRODUCT_DEFINITION_SHAPE('',$,#16981);
#16917=SHAPE_REPRESENTATION('',(#9624),#16622);
#16973=PRODUCT_DEFINITION_CONTEXT('part definition',#17164,'design');
#16981=PRODUCT_DEFINITION('Horizontal shaft support',
'Horizontal shaft support',#17044,#16973);
#17044=PRODUCT_DEFINITION_FORMATION('',$,#17173);
#17164=APPLICATION_CONTEXT(
'Core Data for Automotive Mechanical Design Process');
#17165=PRODUCT_CONTEXT('part definition',#17164,'mechanical');
#17173=PRODUCT('Horizontal shaft support','Horizontal shaft support',
'Horizontal shaft support',(#17165));
#17285=COLOUR_RGB('Grey',0.48,0.52,0.57);
#17286=FILL_AREA_STYLE_COLOUR('',#17285);
#17287=FILL_AREA_STYLE('',(#17286));
#17288=SURFACE_STYLE_FILL_AREA(#17287);
#17289=SURFACE_SIDE_STYLE('',(#17288));
#17290=SURFACE_STYLE_USAGE(.BOTH.,#17289);
#17291=PRESENTATION_STYLE_ASSIGNMENT((#17290));
ENDSEC;
END-ISO-10303-21;
